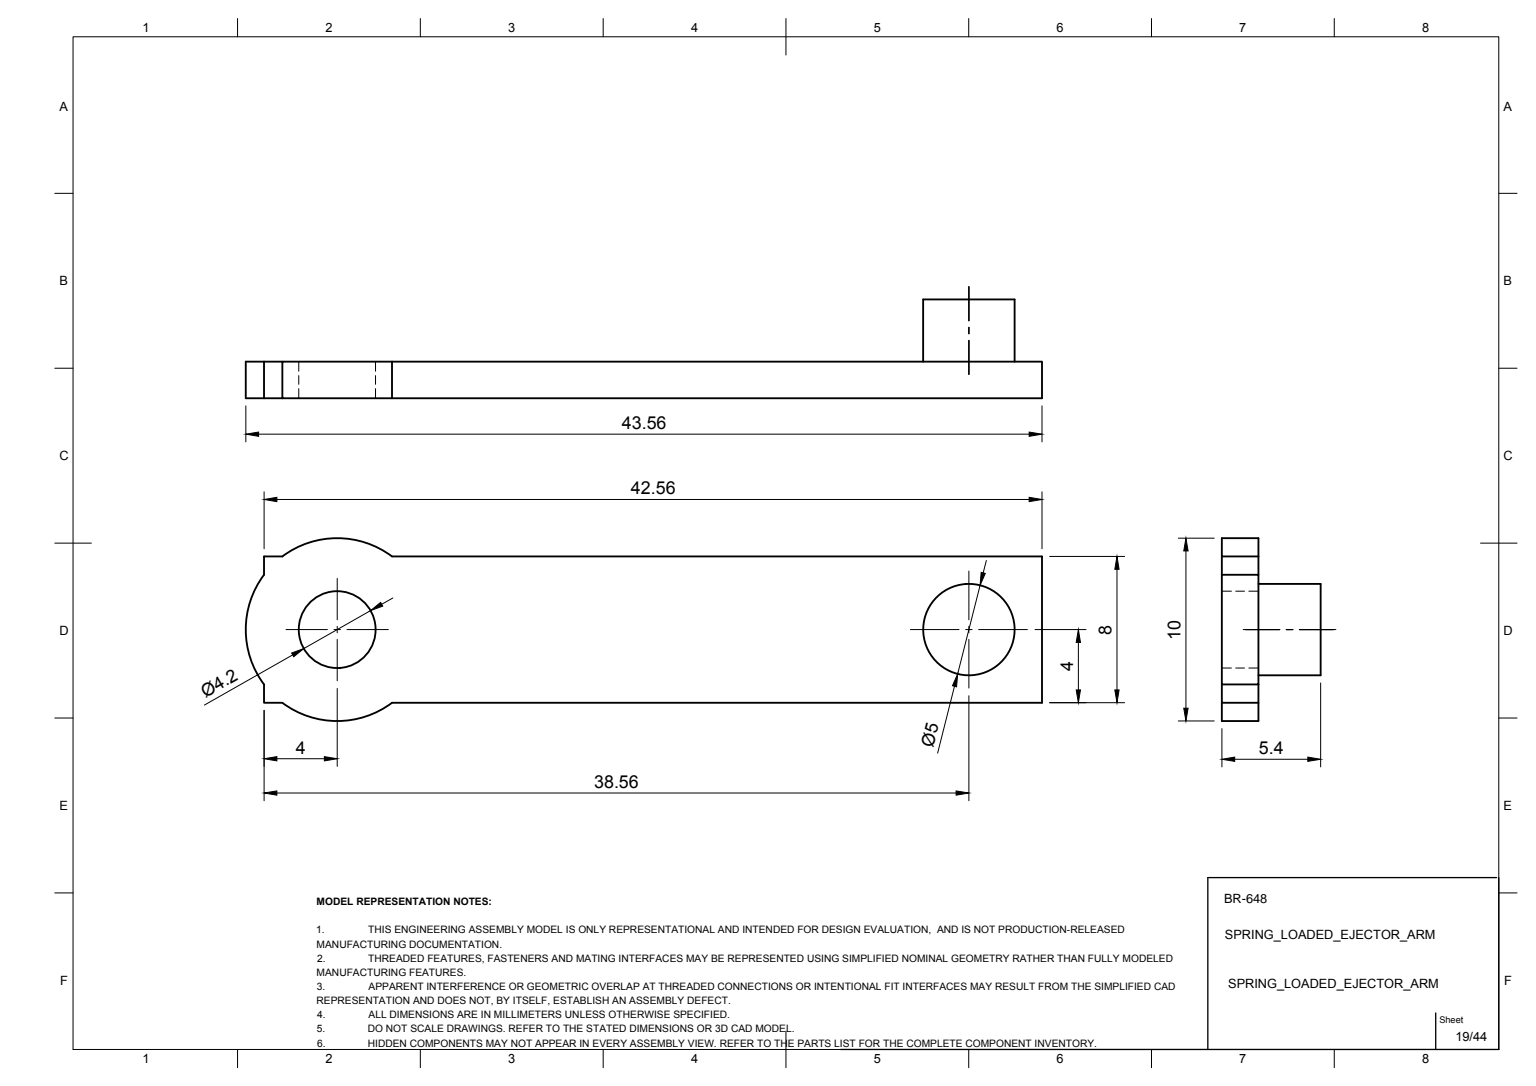
ISO-10303-21;
HEADER;
FILE_DESCRIPTION((''),'2;1');
FILE_NAME('SPRING_LOADED_EJECTOR_ARM.step','2026-10-01T22:05:39-07:00',(''),(''),'','','');
FILE_SCHEMA (('AUTOMOTIVE_DESIGN { 1 0 10303 214 3 1 1 }'));
ENDSEC;
DATA;
#10=MECHANICAL_DESIGN_GEOMETRIC_PRESENTATION_REPRESENTATION('',(#619),#24628);
#535=SHAPE_REPRESENTATION_RELATIONSHIP('SRR','None',#24807,#577) ;
#577=ADVANCED_BREP_SHAPE_REPRESENTATION('',(#659),#24597) ;
#619=STYLED_ITEM('',(#25034),#659) ;
#659=MANIFOLD_SOLID_BREP('SPRING_LOADED_EJECTOR_ARM',#13130) ;
#854=FACE_BOUND('',#4171,.T.) ;
#855=FACE_BOUND('',#4175,.T.) ;
#856=FACE_BOUND('',#4176,.T.) ;
#1329=LINE('',#21129,#2165) ;
#1330=LINE('',#21136,#2166) ;
#1331=LINE('',#21141,#2167) ;
#1332=LINE('',#21145,#2168) ;
#1333=LINE('',#21150,#2169) ;
#1334=LINE('',#21154,#2170) ;
#1335=LINE('',#21159,#2171) ;
#1336=LINE('',#21163,#2172) ;
#1337=LINE('',#21167,#2173) ;
#1338=LINE('',#21169,#2174) ;
#1339=LINE('',#21170,#2175) ;
#1340=LINE('',#21173,#2176) ;
#1341=LINE('',#21175,#2177) ;
#1342=LINE('',#21176,#2178) ;
#1343=LINE('',#21179,#2179) ;
#1344=LINE('',#21181,#2180) ;
#1345=LINE('',#21182,#2181) ;
#1346=LINE('',#21184,#2182) ;
#1347=LINE('',#21186,#2183) ;
#1348=LINE('',#21187,#2184) ;
#1349=LINE('',#21188,#2185) ;
#1350=LINE('',#21190,#2186) ;
#1351=LINE('',#21193,#2187) ;
#1352=LINE('',#21194,#2188) ;
#1353=LINE('',#21196,#2189) ;
#1354=LINE('',#21197,#2190) ;
#2165=VECTOR('',#16874,0.25) ;
#2166=VECTOR('',#16883,0.21) ;
#2167=VECTOR('',#16888,1.) ;
#2168=VECTOR('',#16891,1.) ;
#2169=VECTOR('',#16896,1.) ;
#2170=VECTOR('',#16899,1.) ;
#2171=VECTOR('',#16904,1.) ;
#2172=VECTOR('',#16907,1.) ;
#2173=VECTOR('',#16912,1.) ;
#2174=VECTOR('',#16913,1.) ;
#2175=VECTOR('',#16914,1.) ;
#2176=VECTOR('',#16917,1.) ;
#2177=VECTOR('',#16918,1.) ;
#2178=VECTOR('',#16919,1.) ;
#2179=VECTOR('',#16922,1.) ;
#2180=VECTOR('',#16923,1.) ;
#2181=VECTOR('',#16924,1.) ;
#2182=VECTOR('',#16927,1.) ;
#2183=VECTOR('',#16928,1.) ;
#2184=VECTOR('',#16929,1.) ;
#2185=VECTOR('',#16930,1.) ;
#2186=VECTOR('',#16933,1.) ;
#2187=VECTOR('',#16936,1.) ;
#2188=VECTOR('',#16937,1.) ;
#2189=VECTOR('',#16940,1.) ;
#2190=VECTOR('',#16941,1.) ;
#2806=CYLINDRICAL_SURFACE('',#14228,0.25) ;
#2807=CYLINDRICAL_SURFACE('',#14232,0.21) ;
#2808=CYLINDRICAL_SURFACE('',#14235,0.5) ;
#2809=CYLINDRICAL_SURFACE('',#14238,0.5) ;
#2810=CYLINDRICAL_SURFACE('',#14241,0.5) ;
#3226=FACE_OUTER_BOUND('',#4161,.T.) ;
#3227=FACE_OUTER_BOUND('',#4162,.T.) ;
#3228=FACE_OUTER_BOUND('',#4163,.T.) ;
#3229=FACE_OUTER_BOUND('',#4164,.T.) ;
#3230=FACE_OUTER_BOUND('',#4165,.T.) ;
#3231=FACE_OUTER_BOUND('',#4166,.T.) ;
#3232=FACE_OUTER_BOUND('',#4167,.T.) ;
#3233=FACE_OUTER_BOUND('',#4168,.T.) ;
#3234=FACE_OUTER_BOUND('',#4169,.T.) ;
#3235=FACE_OUTER_BOUND('',#4170,.T.) ;
#3236=FACE_OUTER_BOUND('',#4172,.T.) ;
#3237=FACE_OUTER_BOUND('',#4173,.T.) ;
#3238=FACE_OUTER_BOUND('',#4174,.T.) ;
#3239=FACE_OUTER_BOUND('',#4177,.T.) ;
#3240=FACE_OUTER_BOUND('',#4178,.T.) ;
#4161=EDGE_LOOP('',(#9723,#9724,#9725,#9726)) ;
#4162=EDGE_LOOP('',(#9727)) ;
#4163=EDGE_LOOP('',(#9728,#9729,#9730,#9731)) ;
#4164=EDGE_LOOP('',(#9732,#9733,#9734,#9735)) ;
#4165=EDGE_LOOP('',(#9736,#9737,#9738,#9739)) ;
#4166=EDGE_LOOP('',(#9740,#9741,#9742,#9743)) ;
#4167=EDGE_LOOP('',(#9744,#9745,#9746,#9747)) ;
#4168=EDGE_LOOP('',(#9748,#9749,#9750,#9751)) ;
#4169=EDGE_LOOP('',(#9752,#9753,#9754,#9755)) ;
#4170=EDGE_LOOP('',(#9756,#9757,#9758,#9759,#9760,#9761,#9762,#9763,#9764,
#9765)) ;
#4171=EDGE_LOOP('',(#9766)) ;
#4172=EDGE_LOOP('',(#9767,#9768,#9769,#9770)) ;
#4173=EDGE_LOOP('',(#9771,#9772,#9773,#9774)) ;
#4174=EDGE_LOOP('',(#9775,#9776,#9777,#9778,#9779,#9780,#9781,#9782,#9783,
#9784)) ;
#4175=EDGE_LOOP('',(#9785)) ;
#4176=EDGE_LOOP('',(#9786)) ;
#4177=EDGE_LOOP('',(#9787,#9788,#9789,#9790)) ;
#4178=EDGE_LOOP('',(#9791,#9792,#9793,#9794)) ;
#5036=CIRCLE('',#14229,0.25) ;
#5037=CIRCLE('',#14230,0.25) ;
#5038=CIRCLE('',#14233,0.21) ;
#5039=CIRCLE('',#14234,0.21) ;
#5040=CIRCLE('',#14236,0.5) ;
#5041=CIRCLE('',#14237,0.5) ;
#5042=CIRCLE('',#14239,0.5) ;
#5043=CIRCLE('',#14240,0.5) ;
#5044=CIRCLE('',#14242,0.5) ;
#5045=CIRCLE('',#14243,0.5) ;
#5949=VERTEX_POINT('',#21126) ;
#5950=VERTEX_POINT('',#21128) ;
#5951=VERTEX_POINT('',#21133) ;
#5952=VERTEX_POINT('',#21135) ;
#5953=VERTEX_POINT('',#21139) ;
#5954=VERTEX_POINT('',#21140) ;
#5955=VERTEX_POINT('',#21142) ;
#5956=VERTEX_POINT('',#21144) ;
#5957=VERTEX_POINT('',#21148) ;
#5958=VERTEX_POINT('',#21149) ;
#5959=VERTEX_POINT('',#21151) ;
#5960=VERTEX_POINT('',#21153) ;
#5961=VERTEX_POINT('',#21157) ;
#5962=VERTEX_POINT('',#21158) ;
#5963=VERTEX_POINT('',#21160) ;
#5964=VERTEX_POINT('',#21162) ;
#5965=VERTEX_POINT('',#21166) ;
#5966=VERTEX_POINT('',#21168) ;
#5967=VERTEX_POINT('',#21172) ;
#5968=VERTEX_POINT('',#21174) ;
#5969=VERTEX_POINT('',#21178) ;
#5970=VERTEX_POINT('',#21180) ;
#5971=VERTEX_POINT('',#21185) ;
#5972=VERTEX_POINT('',#21192) ;
#7351=EDGE_CURVE('',#5949,#5949,#5036,.T.) ;
#7352=EDGE_CURVE('',#5949,#5950,#1329,.T.) ;
#7353=EDGE_CURVE('',#5950,#5950,#5037,.T.) ;
#7354=EDGE_CURVE('',#5951,#5951,#5038,.T.) ;
#7355=EDGE_CURVE('',#5951,#5952,#1330,.T.) ;
#7356=EDGE_CURVE('',#5952,#5952,#5039,.T.) ;
#7357=EDGE_CURVE('',#5953,#5954,#1331,.T.) ;
#7358=EDGE_CURVE('',#5955,#5953,#5040,.T.) ;
#7359=EDGE_CURVE('',#5956,#5955,#1332,.T.) ;
#7360=EDGE_CURVE('',#5954,#5956,#5041,.T.) ;
#7361=EDGE_CURVE('',#5957,#5958,#1333,.T.) ;
#7362=EDGE_CURVE('',#5959,#5957,#5042,.T.) ;
#7363=EDGE_CURVE('',#5960,#5959,#1334,.T.) ;
#7364=EDGE_CURVE('',#5958,#5960,#5043,.T.) ;
#7365=EDGE_CURVE('',#5961,#5962,#1335,.T.) ;
#7366=EDGE_CURVE('',#5963,#5961,#5044,.T.) ;
#7367=EDGE_CURVE('',#5964,#5963,#1336,.T.) ;
#7368=EDGE_CURVE('',#5962,#5964,#5045,.T.) ;
#7369=EDGE_CURVE('',#5963,#5965,#1337,.T.) ;
#7370=EDGE_CURVE('',#5965,#5966,#1338,.T.) ;
#7371=EDGE_CURVE('',#5966,#5964,#1339,.T.) ;
#7372=EDGE_CURVE('',#5962,#5967,#1340,.T.) ;
#7373=EDGE_CURVE('',#5967,#5968,#1341,.T.) ;
#7374=EDGE_CURVE('',#5968,#5961,#1342,.T.) ;
#7375=EDGE_CURVE('',#5959,#5969,#1343,.T.) ;
#7376=EDGE_CURVE('',#5970,#5969,#1344,.T.) ;
#7377=EDGE_CURVE('',#5960,#5970,#1345,.T.) ;
#7378=EDGE_CURVE('',#5967,#5957,#1346,.T.) ;
#7379=EDGE_CURVE('',#5966,#5971,#1347,.T.) ;
#7380=EDGE_CURVE('',#5954,#5971,#1348,.T.) ;
#7381=EDGE_CURVE('',#5969,#5956,#1349,.T.) ;
#7382=EDGE_CURVE('',#5955,#5970,#1350,.T.) ;
#7383=EDGE_CURVE('',#5971,#5972,#1351,.T.) ;
#7384=EDGE_CURVE('',#5972,#5953,#1352,.T.) ;
#7385=EDGE_CURVE('',#5968,#5958,#1353,.T.) ;
#7386=EDGE_CURVE('',#5965,#5972,#1354,.T.) ;
#9723=ORIENTED_EDGE('',*,*,#7351,.F.) ;
#9724=ORIENTED_EDGE('',*,*,#7352,.T.) ;
#9725=ORIENTED_EDGE('',*,*,#7353,.F.) ;
#9726=ORIENTED_EDGE('',*,*,#7352,.F.) ;
#9727=ORIENTED_EDGE('',*,*,#7353,.T.) ;
#9728=ORIENTED_EDGE('',*,*,#7354,.F.) ;
#9729=ORIENTED_EDGE('',*,*,#7355,.T.) ;
#9730=ORIENTED_EDGE('',*,*,#7356,.F.) ;
#9731=ORIENTED_EDGE('',*,*,#7355,.F.) ;
#9732=ORIENTED_EDGE('',*,*,#7357,.F.) ;
#9733=ORIENTED_EDGE('',*,*,#7358,.F.) ;
#9734=ORIENTED_EDGE('',*,*,#7359,.F.) ;
#9735=ORIENTED_EDGE('',*,*,#7360,.F.) ;
#9736=ORIENTED_EDGE('',*,*,#7361,.F.) ;
#9737=ORIENTED_EDGE('',*,*,#7362,.F.) ;
#9738=ORIENTED_EDGE('',*,*,#7363,.F.) ;
#9739=ORIENTED_EDGE('',*,*,#7364,.F.) ;
#9740=ORIENTED_EDGE('',*,*,#7365,.F.) ;
#9741=ORIENTED_EDGE('',*,*,#7366,.F.) ;
#9742=ORIENTED_EDGE('',*,*,#7367,.F.) ;
#9743=ORIENTED_EDGE('',*,*,#7368,.F.) ;
#9744=ORIENTED_EDGE('',*,*,#7367,.T.) ;
#9745=ORIENTED_EDGE('',*,*,#7369,.T.) ;
#9746=ORIENTED_EDGE('',*,*,#7370,.T.) ;
#9747=ORIENTED_EDGE('',*,*,#7371,.T.) ;
#9748=ORIENTED_EDGE('',*,*,#7365,.T.) ;
#9749=ORIENTED_EDGE('',*,*,#7372,.T.) ;
#9750=ORIENTED_EDGE('',*,*,#7373,.T.) ;
#9751=ORIENTED_EDGE('',*,*,#7374,.T.) ;
#9752=ORIENTED_EDGE('',*,*,#7363,.T.) ;
#9753=ORIENTED_EDGE('',*,*,#7375,.T.) ;
#9754=ORIENTED_EDGE('',*,*,#7376,.F.) ;
#9755=ORIENTED_EDGE('',*,*,#7377,.F.) ;
#9756=ORIENTED_EDGE('',*,*,#7378,.F.) ;
#9757=ORIENTED_EDGE('',*,*,#7372,.F.) ;
#9758=ORIENTED_EDGE('',*,*,#7368,.T.) ;
#9759=ORIENTED_EDGE('',*,*,#7371,.F.) ;
#9760=ORIENTED_EDGE('',*,*,#7379,.T.) ;
#9761=ORIENTED_EDGE('',*,*,#7380,.F.) ;
#9762=ORIENTED_EDGE('',*,*,#7360,.T.) ;
#9763=ORIENTED_EDGE('',*,*,#7381,.F.) ;
#9764=ORIENTED_EDGE('',*,*,#7375,.F.) ;
#9765=ORIENTED_EDGE('',*,*,#7362,.T.) ;
#9766=ORIENTED_EDGE('',*,*,#7356,.T.) ;
#9767=ORIENTED_EDGE('',*,*,#7359,.T.) ;
#9768=ORIENTED_EDGE('',*,*,#7382,.T.) ;
#9769=ORIENTED_EDGE('',*,*,#7376,.T.) ;
#9770=ORIENTED_EDGE('',*,*,#7381,.T.) ;
#9771=ORIENTED_EDGE('',*,*,#7357,.T.) ;
#9772=ORIENTED_EDGE('',*,*,#7380,.T.) ;
#9773=ORIENTED_EDGE('',*,*,#7383,.T.) ;
#9774=ORIENTED_EDGE('',*,*,#7384,.T.) ;
#9775=ORIENTED_EDGE('',*,*,#7374,.F.) ;
#9776=ORIENTED_EDGE('',*,*,#7385,.T.) ;
#9777=ORIENTED_EDGE('',*,*,#7364,.T.) ;
#9778=ORIENTED_EDGE('',*,*,#7377,.T.) ;
#9779=ORIENTED_EDGE('',*,*,#7382,.F.) ;
#9780=ORIENTED_EDGE('',*,*,#7358,.T.) ;
#9781=ORIENTED_EDGE('',*,*,#7384,.F.) ;
#9782=ORIENTED_EDGE('',*,*,#7386,.F.) ;
#9783=ORIENTED_EDGE('',*,*,#7369,.F.) ;
#9784=ORIENTED_EDGE('',*,*,#7366,.T.) ;
#9785=ORIENTED_EDGE('',*,*,#7351,.T.) ;
#9786=ORIENTED_EDGE('',*,*,#7354,.T.) ;
#9787=ORIENTED_EDGE('',*,*,#7361,.T.) ;
#9788=ORIENTED_EDGE('',*,*,#7385,.F.) ;
#9789=ORIENTED_EDGE('',*,*,#7373,.F.) ;
#9790=ORIENTED_EDGE('',*,*,#7378,.T.) ;
#9791=ORIENTED_EDGE('',*,*,#7386,.T.) ;
#9792=ORIENTED_EDGE('',*,*,#7383,.F.) ;
#9793=ORIENTED_EDGE('',*,*,#7379,.F.) ;
#9794=ORIENTED_EDGE('',*,*,#7370,.F.) ;
#12136=PLANE('',#14231) ;
#12137=PLANE('',#14244) ;
#12138=PLANE('',#14245) ;
#12139=PLANE('',#14246) ;
#12140=PLANE('',#14247) ;
#12141=PLANE('',#14248) ;
#12142=PLANE('',#14249) ;
#12143=PLANE('',#14250) ;
#12144=PLANE('',#14251) ;
#12145=PLANE('',#14252) ;
#12621=ADVANCED_FACE('',(#3226),#2806,.T.) ;
#12622=ADVANCED_FACE('',(#3227),#12136,.T.) ;
#12623=ADVANCED_FACE('',(#3228),#2807,.F.) ;
#12624=ADVANCED_FACE('',(#3229),#2808,.T.) ;
#12625=ADVANCED_FACE('',(#3230),#2809,.T.) ;
#12626=ADVANCED_FACE('',(#3231),#2810,.T.) ;
#12627=ADVANCED_FACE('',(#3232),#12137,.T.) ;
#12628=ADVANCED_FACE('',(#3233),#12138,.T.) ;
#12629=ADVANCED_FACE('',(#3234),#12139,.F.) ;
#12630=ADVANCED_FACE('',(#3235,#854),#12140,.F.) ;
#12631=ADVANCED_FACE('',(#3236),#12141,.F.) ;
#12632=ADVANCED_FACE('',(#3237),#12142,.F.) ;
#12633=ADVANCED_FACE('',(#3238,#855,#856),#12143,.F.) ;
#12634=ADVANCED_FACE('',(#3239),#12144,.F.) ;
#12635=ADVANCED_FACE('',(#3240),#12145,.F.) ;
#13130=CLOSED_SHELL('',(#12621,#12622,#12623,#12624,#12625,#12626,#12627,
#12628,#12629,#12630,#12631,#12632,#12633,#12634,#12635)) ;
#14227=AXIS2_PLACEMENT_3D('',#21124,#16868,#16869) ;
#14228=AXIS2_PLACEMENT_3D('',#21125,#16870,#16871) ;
#14229=AXIS2_PLACEMENT_3D('',#21127,#16872,#16873) ;
#14230=AXIS2_PLACEMENT_3D('',#21130,#16875,#16876) ;
#14231=AXIS2_PLACEMENT_3D('',#21131,#16877,#16878) ;
#14232=AXIS2_PLACEMENT_3D('',#21132,#16879,#16880) ;
#14233=AXIS2_PLACEMENT_3D('',#21134,#16881,#16882) ;
#14234=AXIS2_PLACEMENT_3D('',#21137,#16884,#16885) ;
#14235=AXIS2_PLACEMENT_3D('',#21138,#16886,#16887) ;
#14236=AXIS2_PLACEMENT_3D('',#21143,#16889,#16890) ;
#14237=AXIS2_PLACEMENT_3D('',#21146,#16892,#16893) ;
#14238=AXIS2_PLACEMENT_3D('',#21147,#16894,#16895) ;
#14239=AXIS2_PLACEMENT_3D('',#21152,#16897,#16898) ;
#14240=AXIS2_PLACEMENT_3D('',#21155,#16900,#16901) ;
#14241=AXIS2_PLACEMENT_3D('',#21156,#16902,#16903) ;
#14242=AXIS2_PLACEMENT_3D('',#21161,#16905,#16906) ;
#14243=AXIS2_PLACEMENT_3D('',#21164,#16908,#16909) ;
#14244=AXIS2_PLACEMENT_3D('',#21165,#16910,#16911) ;
#14245=AXIS2_PLACEMENT_3D('',#21171,#16915,#16916) ;
#14246=AXIS2_PLACEMENT_3D('',#21177,#16920,#16921) ;
#14247=AXIS2_PLACEMENT_3D('',#21183,#16925,#16926) ;
#14248=AXIS2_PLACEMENT_3D('',#21189,#16931,#16932) ;
#14249=AXIS2_PLACEMENT_3D('',#21191,#16934,#16935) ;
#14250=AXIS2_PLACEMENT_3D('',#21195,#16938,#16939) ;
#14251=AXIS2_PLACEMENT_3D('',#21198,#16942,#16943) ;
#14252=AXIS2_PLACEMENT_3D('',#21199,#16944,#16945) ;
#16868=DIRECTION('axis',(0.,0.,1.)) ;
#16869=DIRECTION('refdir',(1.,0.,0.)) ;
#16870=DIRECTION('center_axis',(0.,1.,0.)) ;
#16871=DIRECTION('ref_axis',(1.,0.,0.)) ;
#16872=DIRECTION('center_axis',(0.,1.,0.)) ;
#16873=DIRECTION('ref_axis',(1.,0.,0.)) ;
#16874=DIRECTION('',(0.,-1.,0.)) ;
#16875=DIRECTION('center_axis',(0.,-1.,0.)) ;
#16876=DIRECTION('ref_axis',(1.,0.,0.)) ;
#16877=DIRECTION('center_axis',(0.,-1.,0.)) ;
#16878=DIRECTION('ref_axis',(-1.,0.,0.)) ;
#16879=DIRECTION('center_axis',(0.,1.,0.)) ;
#16880=DIRECTION('ref_axis',(1.,0.,0.)) ;
#16881=DIRECTION('center_axis',(0.,1.,0.)) ;
#16882=DIRECTION('ref_axis',(1.,0.,0.)) ;
#16883=DIRECTION('',(0.,1.,0.)) ;
#16884=DIRECTION('center_axis',(0.,-1.,0.)) ;
#16885=DIRECTION('ref_axis',(1.,0.,0.)) ;
#16886=DIRECTION('center_axis',(0.,1.,0.)) ;
#16887=DIRECTION('ref_axis',(-0.997582534658001,0.,0.0694916293183479)) ;
#16888=DIRECTION('',(0.,1.,0.)) ;
#16889=DIRECTION('center_axis',(0.,-1.,0.)) ;
#16890=DIRECTION('ref_axis',(1.,0.,0.)) ;
#16891=DIRECTION('',(0.,-1.,0.)) ;
#16892=DIRECTION('center_axis',(0.,1.,0.)) ;
#16893=DIRECTION('ref_axis',(1.,0.,0.)) ;
#16894=DIRECTION('center_axis',(0.,1.,0.)) ;
#16895=DIRECTION('ref_axis',(1.,0.,0.)) ;
#16896=DIRECTION('',(0.,-1.,0.)) ;
#16897=DIRECTION('center_axis',(0.,1.,0.)) ;
#16898=DIRECTION('ref_axis',(1.,0.,0.)) ;
#16899=DIRECTION('',(0.,1.,0.)) ;
#16900=DIRECTION('center_axis',(0.,-1.,0.)) ;
#16901=DIRECTION('ref_axis',(1.,0.,0.)) ;
#16902=DIRECTION('center_axis',(0.,1.,0.)) ;
#16903=DIRECTION('ref_axis',(1.,0.,0.)) ;
#16904=DIRECTION('',(0.,1.,0.)) ;
#16905=DIRECTION('center_axis',(0.,-1.,0.)) ;
#16906=DIRECTION('ref_axis',(1.,0.,0.)) ;
#16907=DIRECTION('',(0.,-1.,0.)) ;
#16908=DIRECTION('center_axis',(0.,1.,0.)) ;
#16909=DIRECTION('ref_axis',(1.,0.,0.)) ;
#16910=DIRECTION('center_axis',(0.997582534658001,0.,-0.0694916293183465)) ;
#16911=DIRECTION('ref_axis',(-0.0694916293183465,0.,-0.997582534658001)) ;
#16912=DIRECTION('',(-0.0694916293183465,0.,-0.997582534658001)) ;
#16913=DIRECTION('',(0.,1.,0.)) ;
#16914=DIRECTION('',(0.0694916293183465,0.,0.997582534658001)) ;
#16915=DIRECTION('center_axis',(0.997582534658001,0.,-0.0694916293183465)) ;
#16916=DIRECTION('ref_axis',(-0.0694916293183465,0.,-0.997582534658001)) ;
#16917=DIRECTION('',(0.0694916293183465,0.,0.997582534658001)) ;
#16918=DIRECTION('',(0.,-1.,0.)) ;
#16919=DIRECTION('',(-0.0694916293183465,0.,-0.997582534658001)) ;
#16920=DIRECTION('center_axis',(-0.0694916293183465,0.,-0.997582534658001)) ;
#16921=DIRECTION('ref_axis',(-0.997582534658001,0.,0.0694916293183465)) ;
#16922=DIRECTION('',(-0.997582534658001,0.,0.0694916293183465)) ;
#16923=DIRECTION('',(0.,1.,0.)) ;
#16924=DIRECTION('',(-0.997582534658001,0.,0.0694916293183465)) ;
#16925=DIRECTION('center_axis',(0.,-1.,0.)) ;
#16926=DIRECTION('ref_axis',(-0.997582534658001,0.,0.0694916293183465)) ;
#16927=DIRECTION('',(-0.997582534658001,0.,0.0694916293183465)) ;
#16928=DIRECTION('',(-0.997582534658001,0.,0.0694916293183465)) ;
#16929=DIRECTION('',(-0.0694916293183465,0.,-0.997582534658001)) ;
#16930=DIRECTION('',(-0.0694916293183465,0.,-0.997582534658001)) ;
#16931=DIRECTION('center_axis',(0.997582534658001,0.,-0.0694916293183465)) ;
#16932=DIRECTION('ref_axis',(-0.0694916293183465,0.,-0.997582534658001)) ;
#16933=DIRECTION('',(0.0694916293183465,0.,0.997582534658001)) ;
#16934=DIRECTION('center_axis',(0.997582534658001,0.,-0.0694916293183465)) ;
#16935=DIRECTION('ref_axis',(-0.0694916293183465,0.,-0.997582534658001)) ;
#16936=DIRECTION('',(0.,-1.,0.)) ;
#16937=DIRECTION('',(0.0694916293183465,0.,0.997582534658001)) ;
#16938=DIRECTION('center_axis',(0.,1.,0.)) ;
#16939=DIRECTION('ref_axis',(0.997582534658001,0.,-0.0694916293183465)) ;
#16940=DIRECTION('',(-0.997582534658001,0.,0.0694916293183465)) ;
#16941=DIRECTION('',(-0.997582534658001,0.,0.0694916293183465)) ;
#16942=DIRECTION('center_axis',(-0.0694916293183465,0.,-0.997582534658001)) ;
#16943=DIRECTION('ref_axis',(-0.997582534658001,0.,0.0694916293183465)) ;
#16944=DIRECTION('center_axis',(0.0694916293183465,0.,0.997582534658001)) ;
#16945=DIRECTION('ref_axis',(0.997582534658001,0.,-0.0694916293183465)) ;
#21124=CARTESIAN_POINT('',(0.,0.,0.)) ;
#21125=CARTESIAN_POINT('Origin',(-6.43477332219942,-0.07,5.39941592136693)) ;
#21126=CARTESIAN_POINT('',(-6.68477332219942,0.1,5.39941592136693)) ;
#21127=CARTESIAN_POINT('Origin',(-6.43477332219942,0.1,5.39941592136693)) ;
#21128=CARTESIAN_POINT('',(-6.68477332219942,-0.24,5.39941592136693)) ;
#21129=CARTESIAN_POINT('',(-6.68477332219942,-0.07,5.39941592136693)) ;
#21130=CARTESIAN_POINT('Origin',(-6.43477332219942,-0.24,5.39941592136693)) ;
#21131=CARTESIAN_POINT('Origin',(-6.43477332219942,-0.24,5.39941592136693)) ;
#21132=CARTESIAN_POINT('Origin',(-6.1946255125913,0.2,8.84684207832111)) ;
#21133=CARTESIAN_POINT('',(-6.4046255125913,0.1,8.84684207832111)) ;
#21134=CARTESIAN_POINT('Origin',(-6.1946255125913,0.1,8.84684207832111)) ;
#21135=CARTESIAN_POINT('',(-6.4046255125913,0.3,8.84684207832111)) ;
#21136=CARTESIAN_POINT('',(-6.4046255125913,0.2,8.84684207832111)) ;
#21137=CARTESIAN_POINT('Origin',(-6.1946255125913,0.3,8.84684207832111)) ;
#21138=CARTESIAN_POINT('Origin',(-6.1946255125913,0.2,8.84684207832111)) ;
#21139=CARTESIAN_POINT('',(-6.61450601525,0.1,8.57536396965105)) ;
#21140=CARTESIAN_POINT('',(-6.61450601525,0.3,8.57536396965105)) ;
#21141=CARTESIAN_POINT('',(-6.61450601525,0.2,8.57536396965105)) ;
#21142=CARTESIAN_POINT('',(-6.57281103765899,0.1,9.17391349044585)) ;
#21143=CARTESIAN_POINT('Origin',(-6.1946255125913,0.1,8.84684207832111)) ;
#21144=CARTESIAN_POINT('',(-6.57281103765899,0.3,9.17391349044585)) ;
#21145=CARTESIAN_POINT('',(-6.57281103765899,0.2,9.17391349044585)) ;
#21146=CARTESIAN_POINT('Origin',(-6.1946255125913,0.3,8.84684207832111)) ;
#21147=CARTESIAN_POINT('Origin',(-6.1946255125913,0.2,8.84684207832111)) ;
#21148=CARTESIAN_POINT('',(-5.86755410046656,0.3,9.22502760338881)) ;
#21149=CARTESIAN_POINT('',(-5.86755410046656,0.1,9.22502760338881)) ;
#21150=CARTESIAN_POINT('',(-5.86755410046656,0.2,9.22502760338881)) ;
#21151=CARTESIAN_POINT('',(-6.46610362126136,0.3,9.26672258097981)) ;
#21152=CARTESIAN_POINT('Origin',(-6.1946255125913,0.3,8.84684207832111)) ;
#21153=CARTESIAN_POINT('',(-6.46610362126136,0.1,9.26672258097981)) ;
#21154=CARTESIAN_POINT('',(-6.46610362126136,0.2,9.26672258097981)) ;
#21155=CARTESIAN_POINT('Origin',(-6.1946255125913,0.1,8.84684207832111)) ;
#21156=CARTESIAN_POINT('Origin',(-6.1946255125913,0.2,8.84684207832111)) ;
#21157=CARTESIAN_POINT('',(-5.77474500993259,0.1,9.11832018699117)) ;
#21158=CARTESIAN_POINT('',(-5.77474500993259,0.3,9.11832018699117)) ;
#21159=CARTESIAN_POINT('',(-5.77474500993259,0.2,9.11832018699117)) ;
#21160=CARTESIAN_POINT('',(-5.8164399875236,0.1,8.51977066619637)) ;
#21161=CARTESIAN_POINT('Origin',(-6.1946255125913,0.1,8.84684207832111)) ;
#21162=CARTESIAN_POINT('',(-5.8164399875236,0.3,8.51977066619637)) ;
#21163=CARTESIAN_POINT('',(-5.8164399875236,0.2,8.51977066619637)) ;
#21164=CARTESIAN_POINT('Origin',(-6.1946255125913,0.3,8.84684207832111)) ;
#21165=CARTESIAN_POINT('Origin',(-5.91566640353216,0.2,7.09533234811668)) ;
#21166=CARTESIAN_POINT('',(-6.06353696006355,0.1,4.97258625577639)) ;
#21167=CARTESIAN_POINT('',(-5.91566640353216,0.1,7.09533234811668)) ;
#21168=CARTESIAN_POINT('',(-6.06353696006355,0.3,4.97258625577639)) ;
#21169=CARTESIAN_POINT('',(-6.06353696006355,0.2,4.97258625577639)) ;
#21170=CARTESIAN_POINT('',(-5.91566640353216,0.3,7.09533234811668)) ;
#21171=CARTESIAN_POINT('Origin',(-5.91566640353216,0.2,7.09533234811668)) ;
#21172=CARTESIAN_POINT('',(-5.76779584700076,0.3,9.21807844045697)) ;
#21173=CARTESIAN_POINT('',(-5.91566640353216,0.3,7.09533234811668)) ;
#21174=CARTESIAN_POINT('',(-5.76779584700076,0.1,9.21807844045697)) ;
#21175=CARTESIAN_POINT('',(-5.76779584700076,0.2,9.21807844045697)) ;
#21176=CARTESIAN_POINT('',(-5.91566640353216,0.1,7.09533234811668)) ;
#21177=CARTESIAN_POINT('Origin',(-6.16682886086396,0.2,9.24587509218431)) ;
#21178=CARTESIAN_POINT('',(-6.56586187472716,0.3,9.27367174391165)) ;
#21179=CARTESIAN_POINT('',(-6.16682886086396,0.3,9.24587509218431)) ;
#21180=CARTESIAN_POINT('',(-6.56586187472716,0.1,9.27367174391165)) ;
#21181=CARTESIAN_POINT('',(-6.56586187472716,0.2,9.27367174391165)) ;
#21182=CARTESIAN_POINT('',(-6.16682886086396,0.1,9.24587509218431)) ;
#21183=CARTESIAN_POINT('Origin',(-6.31469941739536,0.3,7.12312899984402)) ;
#21184=CARTESIAN_POINT('',(-6.16682886086396,0.3,9.24587509218431)) ;
#21185=CARTESIAN_POINT('',(-6.86160298778995,0.3,5.02817955923107)) ;
#21186=CARTESIAN_POINT('',(-6.46256997392675,0.3,5.00038290750373)) ;
#21187=CARTESIAN_POINT('',(-6.71373243125856,0.3,7.15092565157136)) ;
#21188=CARTESIAN_POINT('',(-6.71373243125856,0.3,7.15092565157136)) ;
#21189=CARTESIAN_POINT('Origin',(-6.71373243125856,0.2,7.15092565157136)) ;
#21190=CARTESIAN_POINT('',(-6.71373243125856,0.1,7.15092565157136)) ;
#21191=CARTESIAN_POINT('Origin',(-6.71373243125856,0.2,7.15092565157136)) ;
#21192=CARTESIAN_POINT('',(-6.86160298778995,0.1,5.02817955923107)) ;
#21193=CARTESIAN_POINT('',(-6.86160298778995,0.2,5.02817955923107)) ;
#21194=CARTESIAN_POINT('',(-6.71373243125856,0.1,7.15092565157136)) ;
#21195=CARTESIAN_POINT('Origin',(-6.31469941739536,0.1,7.12312899984402)) ;
#21196=CARTESIAN_POINT('',(-6.16682886086396,0.1,9.24587509218431)) ;
#21197=CARTESIAN_POINT('',(-6.46256997392675,0.1,5.00038290750373)) ;
#21198=CARTESIAN_POINT('Origin',(-6.16682886086396,0.2,9.24587509218431)) ;
#21199=CARTESIAN_POINT('Origin',(-6.46256997392675,0.2,5.00038290750373)) ;
#24549=UNCERTAINTY_MEASURE_WITH_UNIT(LENGTH_MEASURE(0.001),#24629,
'DISTANCE_ACCURACY_VALUE',
'Maximum model space distance between geometric entities at asserted c
onnectivities') ;
#24580=UNCERTAINTY_MEASURE_WITH_UNIT(LENGTH_MEASURE(0.001),#24629,
'DISTANCE_ACCURACY_VALUE',
'Maximum model space distance between geometric entities at asserted c
onnectivities') ;
#24597=(
GEOMETRIC_REPRESENTATION_CONTEXT(3)
GLOBAL_UNCERTAINTY_ASSIGNED_CONTEXT((#24549))
GLOBAL_UNIT_ASSIGNED_CONTEXT((#24629,#24631,#24632))
REPRESENTATION_CONTEXT('','3D')
) ;
#24628=(
GEOMETRIC_REPRESENTATION_CONTEXT(3)
GLOBAL_UNCERTAINTY_ASSIGNED_CONTEXT((#24580))
GLOBAL_UNIT_ASSIGNED_CONTEXT((#24629,#24631,#24632))
REPRESENTATION_CONTEXT('','3D')
) ;
#24629=(
LENGTH_UNIT()
NAMED_UNIT(*)
SI_UNIT(.CENTI.,.METRE.)
) ;
#24631=(
NAMED_UNIT(*)
PLANE_ANGLE_UNIT()
SI_UNIT($,.RADIAN.)
) ;
#24632=(
NAMED_UNIT(*)
SI_UNIT($,.STERADIAN.)
SOLID_ANGLE_UNIT()
) ;
#24649=SHAPE_DEFINITION_REPRESENTATION(#24696,#24807) ;
#24696=PRODUCT_DEFINITION_SHAPE('',$,#24855) ;
#24807=SHAPE_REPRESENTATION('',(#14227),#24597) ;
#24838=PRODUCT_DEFINITION_CONTEXT('part definition',#24981,'design') ;
#24855=PRODUCT_DEFINITION('SPRING_LOADED_EJECTOR_ARM',
'SPRING_LOADED_EJECTOR_ARM',#24902,#24838) ;
#24902=PRODUCT_DEFINITION_FORMATION('',$,#24999) ;
#24981=APPLICATION_CONTEXT(
'Core Data for Automotive Mechanical Design Process') ;
#24982=PRODUCT_CONTEXT('part definition',#24981,'mechanical') ;
#24999=PRODUCT('SPRING_LOADED_EJECTOR_ARM','SPRING_LOADED_EJECTOR_ARM',$,
(#24982)) ;
#25034=PRESENTATION_STYLE_ASSIGNMENT((#25044)) ;
#25044=SURFACE_STYLE_USAGE(.BOTH.,#25054) ;
#25054=SURFACE_SIDE_STYLE('',(#25064)) ;
#25064=SURFACE_STYLE_FILL_AREA(#25074) ;
#25074=FILL_AREA_STYLE('Stainless Steel - Satin',(#25084)) ;
#25084=FILL_AREA_STYLE_COLOUR('Stainless Steel - Satin',#25094) ;
#25094=COLOUR_RGB('Stainless Steel - Satin', 0.31764706, 0.68627451, 0.89019608) ;
ENDSEC;
END-ISO-10303-21;
